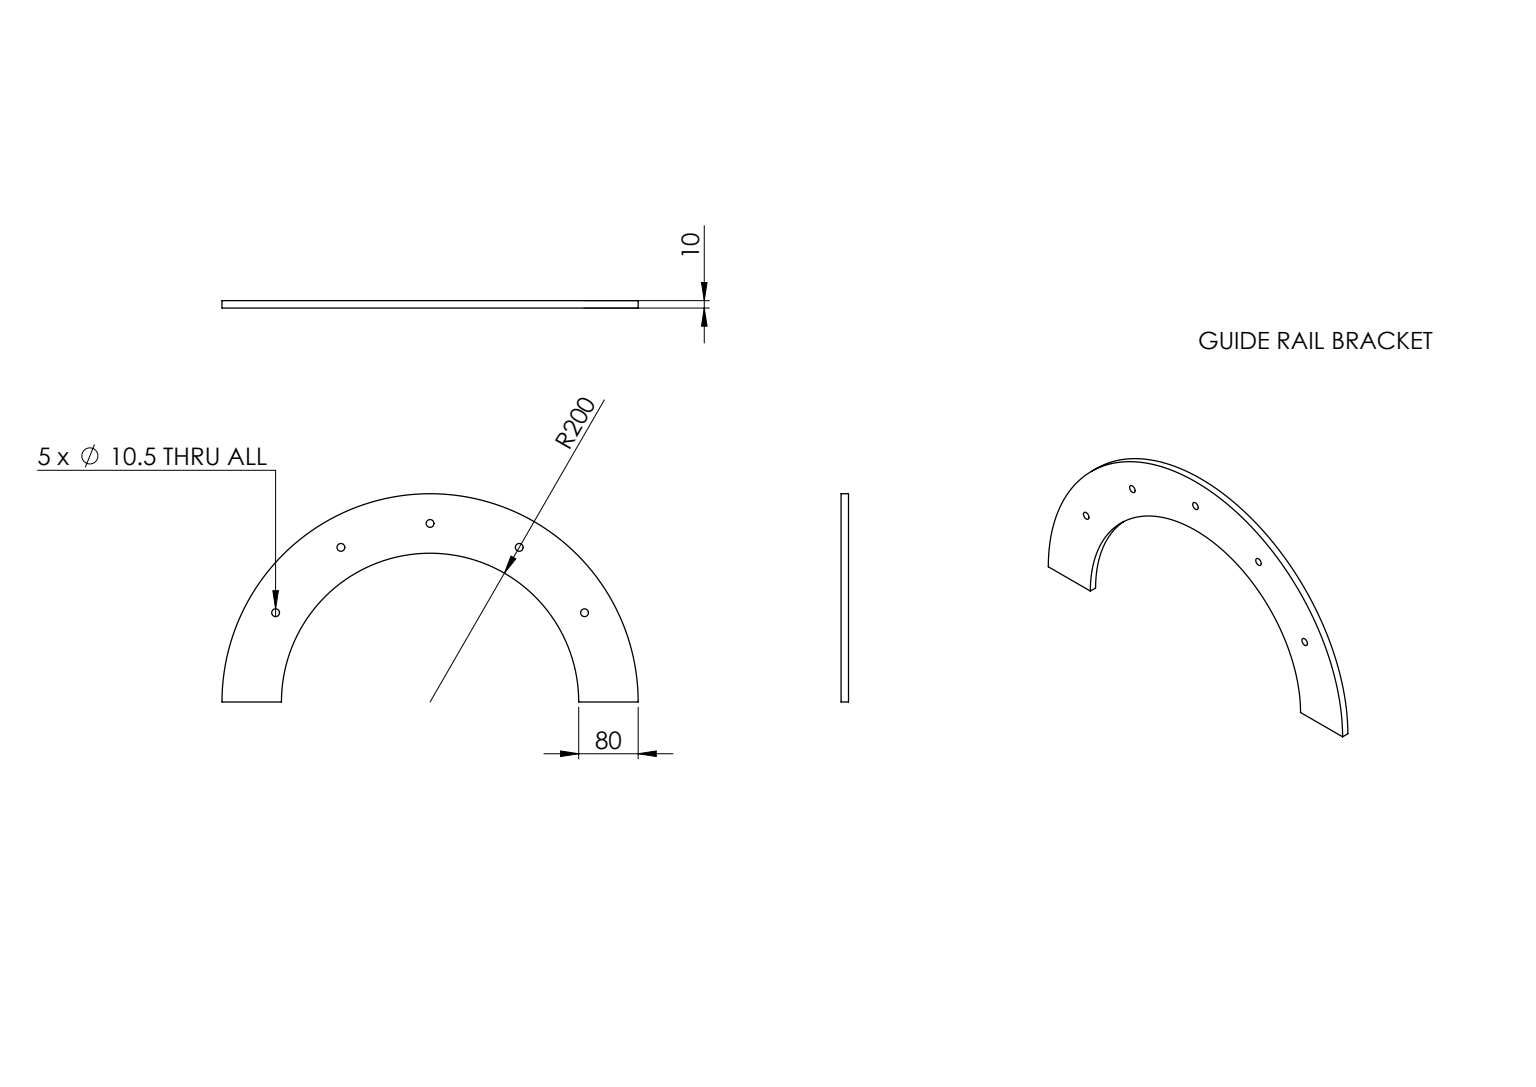
ISO-10303-21;
HEADER;
FILE_DESCRIPTION (('STEP AP214'),
    '1' );
FILE_NAME ('Guide Rail Bracket.step',
    '2026-10-23T05:12:30',
    ( '' ),
    ( '' ),
    'SwSTEP 2.0',
    'SolidWorks 2026',
    '' );
FILE_SCHEMA (( 'AUTOMOTIVE_DESIGN' ));
ENDSEC;

DATA;
#10=CARTESIAN_POINT ( 'NONE',  ( 213.0929183184020701, 119.9981648402868331, 10.00000000000000000 ) ) ;
#18=CARTESIAN_POINT ( 'NONE',  ( -5.249999999999968026, 239.9963296805737230, 10.00000000000000000 ) ) ;
#20=DIRECTION ( 'NONE',  ( -1.000000000000000000, 0.000000000000000000, 0.000000000000000000 ) ) ;
#21=CARTESIAN_POINT ( 'NONE',  ( -279.9963296805736945, 3.428966089163216048E-14, 0.000000000000000000 ) ) ;
#25=DIRECTION ( 'NONE',  ( -0.000000000000000000, -0.000000000000000000, 1.000000000000000000 ) ) ;
#29=DIRECTION ( 'NONE',  ( -1.000000000000000000, 0.000000000000000000, 0.000000000000000000 ) ) ;
#37=CIRCLE ( 'NONE', #2942, 5.249999999999991118 ) ;
#54=FACE_BOUND ( 'NONE', #7641, .T. ) ;
#72=ORIENTED_EDGE ( 'NONE', *, *, #191, .F. ) ;
#80=ORIENTED_EDGE ( 'NONE', *, *, #2127, .F. ) ;
#86=CARTESIAN_POINT ( 'NONE',  ( 1.469553684752138043E-14, 239.9963296805737230, 10.00000000000000178 ) ) ;
#121=CARTESIAN_POINT ( 'NONE',  ( -125.2481648402867762, 207.8429183184021554, -8.673617379884035472E-15 ) ) ;
#157=VECTOR ( 'NONE', #4793, 1000.000000000000000 ) ;
#162=DIRECTION ( 'NONE',  ( -0.000000000000000000, -0.000000000000000000, 1.000000000000000000 ) ) ;
#172=ORIENTED_EDGE ( 'NONE', *, *, #2324, .T. ) ;
#173=AXIS2_PLACEMENT_3D ( 'NONE', #1594, #994, #5732 ) ;
#191=EDGE_CURVE ( 'NONE', #6189, #4002, #7244, .T. ) ;
#198=AXIS2_PLACEMENT_3D ( 'NONE', #1671, #7152, #4070 ) ;
#201=DIRECTION ( 'NONE',  ( -2.403401228516536951E-14, -1.000000000000000000, 0.000000000000000000 ) ) ;
#272=ORIENTED_EDGE ( 'NONE', *, *, #7163, .T. ) ;
#285=CARTESIAN_POINT ( 'NONE',  ( -207.8429183184020985, 119.9981648402869467, 10.00000000000000178 ) ) ;
#298=CIRCLE ( 'NONE', #1308, 5.249999999999976907 ) ;
#311=CARTESIAN_POINT ( 'NONE',  ( 202.5929183184021269, 119.9981648402868331, 10.00000000000000000 ) ) ;
#315=EDGE_CURVE ( 'NONE', #1373, #3431, #4733, .T. ) ;
#334=ORIENTED_EDGE ( 'NONE', *, *, #2127, .T. ) ;
#346=DIRECTION ( 'NONE',  ( 1.000000000000000000, 0.000000000000000000, 0.000000000000000000 ) ) ;
#360=ORIENTED_EDGE ( 'NONE', *, *, #6201, .F. ) ;
#372=EDGE_LOOP ( 'NONE', ( #1862, #4014 ) ) ;
#378=CARTESIAN_POINT ( 'NONE',  ( -279.9963296805736945, 3.428966089163216048E-14, 10.00000000000000000 ) ) ;
#384=DIRECTION ( 'NONE',  ( -0.000000000000000000, -0.000000000000000000, 1.000000000000000000 ) ) ;
#389=DIRECTION ( 'NONE',  ( -0.000000000000000000, -0.000000000000000000, 1.000000000000000000 ) ) ;
#411=EDGE_CURVE ( 'NONE', #2919, #6189, #1551, .T. ) ;
#423=AXIS2_PLACEMENT_3D ( 'NONE', #6991, #7495, #3952 ) ;
#425=CARTESIAN_POINT ( 'NONE',  ( 119.9981648402868899, 207.8429183184021269, 10.00000000000000000 ) ) ;
#431=ORIENTED_EDGE ( 'NONE', *, *, #935, .T. ) ;
#492=ORIENTED_EDGE ( 'NONE', *, *, #2605, .F. ) ;
#551=ORIENTED_EDGE ( 'NONE', *, *, #3232, .F. ) ;
#557=AXIS2_PLACEMENT_3D ( 'NONE', #5104, #4513, #3373 ) ;
#560=EDGE_CURVE ( 'NONE', #7291, #3873, #1586, .T. ) ;
#594=ORIENTED_EDGE ( 'NONE', *, *, #7692, .T. ) ;
#598=DIRECTION ( 'NONE',  ( 1.000000000000000000, 0.000000000000000000, 0.000000000000000000 ) ) ;
#622=DIRECTION ( 'NONE',  ( 1.000000000000000000, 0.000000000000000000, 0.000000000000000000 ) ) ;
#651=DIRECTION ( 'NONE',  ( -0.000000000000000000, -0.000000000000000000, 1.000000000000000000 ) ) ;
#673=DIRECTION ( 'NONE',  ( -1.000000000000000000, 0.000000000000000000, 0.000000000000000000 ) ) ;
#675=CARTESIAN_POINT ( 'NONE',  ( -279.9963296805736945, 3.428966089163216048E-14, 10.00000000000000000 ) ) ;
#690=DIRECTION ( 'NONE',  ( 1.000000000000000000, 0.000000000000000000, 0.000000000000000000 ) ) ;
#710=ORIENTED_EDGE ( 'NONE', *, *, #4511, .F. ) ;
#712=ADVANCED_FACE ( 'NONE', ( #6130 ), #4936, .T. ) ;
#730=CYLINDRICAL_SURFACE ( 'NONE', #6902, 5.249999999999983125 ) ;
#735=ORIENTED_EDGE ( 'NONE', *, *, #1621, .F. ) ;
#745=ORIENTED_EDGE ( 'NONE', *, *, #3810, .T. ) ;
#774=EDGE_LOOP ( 'NONE', ( #3751, #5530 ) ) ;
#785=DIRECTION ( 'NONE',  ( -0.000000000000000000, -0.000000000000000000, 1.000000000000000000 ) ) ;
#800=CIRCLE ( 'NONE', #1055, 5.249999999999976907 ) ;
#808=COLOUR_RGB ( '',0.8941176470588234615, 0.8941176470588234615, 0.8941176470588234615 ) ;
#813=ORIENTED_EDGE ( 'NONE', *, *, #1830, .T. ) ;
#828=FILL_AREA_STYLE ('',( #863 ) ) ;
#852=ADVANCED_FACE ( 'NONE', ( #869 ), #3838, .T. ) ;
#863=FILL_AREA_STYLE_COLOUR ( '', #808 ) ;
#869=FACE_OUTER_BOUND ( 'NONE', #5970, .T. ) ;
#887=VERTEX_POINT ( 'NONE', #3911 ) ;
#893=DIRECTION ( 'NONE',  ( -0.000000000000000000, -0.000000000000000000, 1.000000000000000000 ) ) ;
#904=ORIENTED_EDGE ( 'NONE', *, *, #5478, .F. ) ;
#913=VERTEX_POINT ( 'NONE', #2307 ) ;
#935=EDGE_CURVE ( 'NONE', #887, #5491, #2493, .T. ) ;
#943=DIRECTION ( 'NONE',  ( 1.000000000000000000, 0.000000000000000000, 0.000000000000000000 ) ) ;
#994=DIRECTION ( 'NONE',  ( -0.000000000000000000, -0.000000000000000000, -1.000000000000000000 ) ) ;
#999=EDGE_LOOP ( 'NONE', ( #3310, #3719, #5793, #4925 ) ) ;
#1050=DIRECTION ( 'NONE',  ( -0.000000000000000000, -0.000000000000000000, 1.000000000000000000 ) ) ;
#1055=AXIS2_PLACEMENT_3D ( 'NONE', #2477, #1994, #6680 ) ;
#1063=EDGE_LOOP ( 'NONE', ( #4829, #3062, #2505, #4842 ) ) ;
#1069=FACE_OUTER_BOUND ( 'NONE', #6626, .T. ) ;
#1075=CARTESIAN_POINT ( 'NONE',  ( -119.9981648402868046, 207.8429183184021554, -8.673617379884035472E-15 ) ) ;
#1100=FACE_BOUND ( 'NONE', #7449, .T. ) ;
#1130=ORIENTED_EDGE ( 'NONE', *, *, #6583, .T. ) ;
#1131=ORIENTED_EDGE ( 'NONE', *, *, #5478, .T. ) ;
#1182=ORIENTED_EDGE ( 'NONE', *, *, #6944, .T. ) ;
#1187=AXIS2_PLACEMENT_3D ( 'NONE', #1075, #5935, #4073 ) ;
#1190=ORIENTED_EDGE ( 'NONE', *, *, #3670, .T. ) ;
#1203=ORIENTED_EDGE ( 'NONE', *, *, #2453, .F. ) ;
#1222=AXIS2_PLACEMENT_3D ( 'NONE', #2444, #7326, #5503 ) ;
#1223=PRODUCT_DEFINITION ( 'UNKNOWN', '', #2441, #6530 ) ;
#1245=CARTESIAN_POINT ( 'NONE',  ( 1.469553684752138043E-14, 239.9963296805737230, 10.00000000000000000 ) ) ;
#1263=DIRECTION ( 'NONE',  ( -0.000000000000000000, -0.000000000000000000, -1.000000000000000000 ) ) ;
#1298=VERTEX_POINT ( 'NONE', #2939 ) ;
#1301=CARTESIAN_POINT ( 'NONE',  ( 0.000000000000000000, 0.000000000000000000, 0.000000000000000000 ) ) ;
#1308=AXIS2_PLACEMENT_3D ( 'NONE', #285, #6411, #2158 ) ;
#1341=LINE ( 'NONE', #675, #2511 ) ;
#1373=VERTEX_POINT ( 'NONE', #5397 ) ;
#1379=( NAMED_UNIT ( * ) PLANE_ANGLE_UNIT ( ) SI_UNIT ( $, .RADIAN. ) );
#1411=AXIS2_PLACEMENT_3D ( 'NONE', #86, #7191, #2390 ) ;
#1474=ADVANCED_FACE ( 'NONE', ( #1733 ), #4045, .F. ) ;
#1490=CIRCLE ( 'NONE', #6533, 5.249999999999976907 ) ;
#1498=SURFACE_STYLE_FILL_AREA ( #828 ) ;
#1518=ADVANCED_FACE ( 'NONE', ( #6141 ), #730, .F. ) ;
#1523=ADVANCED_FACE ( 'NONE', ( #7396 ), #3655, .F. ) ;
#1536=SHAPE_REPRESENTATION_RELATIONSHIP ( 'NONE' , 'NONE' ,  #5768, #1719 ) ;
#1539=DIRECTION ( 'NONE',  ( 1.000000000000000000, 2.398081733190338127E-14, 0.000000000000000000 ) ) ;
#1543=DIRECTION ( 'NONE',  ( -0.000000000000000000, -0.000000000000000000, 1.000000000000000000 ) ) ;
#1547=CYLINDRICAL_SURFACE ( 'NONE', #6081, 5.249999999999976907 ) ;
#1551=LINE ( 'NONE', #5140, #1712 ) ;
#1560=ORIENTED_EDGE ( 'NONE', *, *, #7226, .F. ) ;
#1574=DIRECTION ( 'NONE',  ( -0.000000000000000000, -0.000000000000000000, 1.000000000000000000 ) ) ;
#1582=VERTEX_POINT ( 'NONE', #3732 ) ;
#1586=CIRCLE ( 'NONE', #198, 5.249999999999976907 ) ;
#1594=CARTESIAN_POINT ( 'NONE',  ( 0.000000000000000000, 0.000000000000000000, 0.000000000000000000 ) ) ;
#1609=VERTEX_POINT ( 'NONE', #5430 ) ;
#1615=VECTOR ( 'NONE', #25, 1000.000000000000000 ) ;
#1618=EDGE_LOOP ( 'NONE', ( #1560, #2255, #813, #2345 ) ) ;
#1621=EDGE_CURVE ( 'NONE', #3939, #3350, #6218, .T. ) ;
#1641=AXIS2_PLACEMENT_3D ( 'NONE', #3794, #6045, #3674 ) ;
#1671=CARTESIAN_POINT ( 'NONE',  ( -207.8429183184020985, 119.9981648402869467, -8.673617379884035472E-15 ) ) ;
#1680=ORIENTED_EDGE ( 'NONE', *, *, #7692, .F. ) ;
#1687=AXIS2_PLACEMENT_3D ( 'NONE', #5556, #1936, #1859 ) ;
#1701=DIRECTION ( 'NONE',  ( -0.000000000000000000, 0.000000000000000000, -1.000000000000000000 ) ) ;
#1712=VECTOR ( 'NONE', #6252, 1000.000000000000000 ) ;
#1719=ADVANCED_BREP_SHAPE_REPRESENTATION ( '', ( #3160, #7485 ), #7608 ) ;
#1733=FACE_OUTER_BOUND ( 'NONE', #5351, .T. ) ;
#1737=ORIENTED_EDGE ( 'NONE', *, *, #2729, .F. ) ;
#1774=DIRECTION ( 'NONE',  ( -0.000000000000000000, -0.000000000000000000, 1.000000000000000000 ) ) ;
#1784=CARTESIAN_POINT ( 'NONE',  ( -213.0929183184020701, 119.9981648402869467, -8.673617379884035472E-15 ) ) ;
#1799=DIRECTION ( 'NONE',  ( -0.000000000000000000, -0.000000000000000000, -1.000000000000000000 ) ) ;
#1830=EDGE_CURVE ( 'NONE', #1298, #1609, #4113, .T. ) ;
#1859=DIRECTION ( 'NONE',  ( 1.000000000000000000, 0.000000000000000000, 0.000000000000000000 ) ) ;
#1862=ORIENTED_EDGE ( 'NONE', *, *, #315, .F. ) ;
#1895=( LENGTH_UNIT ( ) NAMED_UNIT ( * ) SI_UNIT ( .MILLI., .METRE. ) );
#1910=DIRECTION ( 'NONE',  ( -0.000000000000000000, -0.000000000000000000, 1.000000000000000000 ) ) ;
#1929=EDGE_CURVE ( 'NONE', #5275, #2430, #5638, .T. ) ;
#1936=DIRECTION ( 'NONE',  ( -0.000000000000000000, -0.000000000000000000, 1.000000000000000000 ) ) ;
#1950=CIRCLE ( 'NONE', #557, 5.249999999999977796 ) ;
#1953=FACE_OUTER_BOUND ( 'NONE', #3916, .T. ) ;
#1975=ADVANCED_FACE ( 'NONE', ( #3140, #3178, #54, #7239, #6173, #6648 ), #4270, .T. ) ;
#1980=CARTESIAN_POINT ( 'NONE',  ( -199.9963296805737230, 0.000000000000000000, 0.000000000000000000 ) ) ;
#1994=DIRECTION ( 'NONE',  ( -0.000000000000000000, -0.000000000000000000, 1.000000000000000000 ) ) ;
#2008=AXIS2_PLACEMENT_3D ( 'NONE', #6798, #785, #2652 ) ;
#2063=( NAMED_UNIT ( * ) SI_UNIT ( $, .STERADIAN. ) SOLID_ANGLE_UNIT ( ) );
#2097=DIRECTION ( 'NONE',  ( 1.000000000000000000, 2.398081733190338127E-14, 0.000000000000000000 ) ) ;
#2098=CLOSED_SHELL ( 'NONE', ( #2595, #3549, #7539, #2215, #6494, #3606, #852, #5190, #712, #7026, #1975, #5173, #1523, #1518, #3847, #1474 ) ) ;
#2127=EDGE_CURVE ( 'NONE', #2919, #6450, #6804, .T. ) ;
#2130=ORIENTED_EDGE ( 'NONE', *, *, #5621, .F. ) ;
#2137=CARTESIAN_POINT ( 'NONE',  ( 114.7481648402869041, 207.8429183184021269, 10.00000000000000000 ) ) ;
#2143=SURFACE_STYLE_USAGE ( .BOTH. , #5641 ) ;
#2156=AXIS2_PLACEMENT_3D ( 'NONE', #5561, #1263, #673 ) ;
#2158=DIRECTION ( 'NONE',  ( 1.000000000000000000, 0.000000000000000000, 0.000000000000000000 ) ) ;
#2173=DIRECTION ( 'NONE',  ( -0.000000000000000000, -0.000000000000000000, 1.000000000000000000 ) ) ;
#2181=CARTESIAN_POINT ( 'NONE',  ( 119.9981648402868899, 207.8429183184021269, 10.00000000000000178 ) ) ;
#2215=ADVANCED_FACE ( 'NONE', ( #7425 ), #4980, .F. ) ;
#2244=EDGE_LOOP ( 'NONE', ( #431, #1190 ) ) ;
#2246=ORIENTED_EDGE ( 'NONE', *, *, #411, .T. ) ;
#2254=AXIS2_PLACEMENT_3D ( 'NONE', #3570, #3998, #5301 ) ;
#2255=ORIENTED_EDGE ( 'NONE', *, *, #5817, .F. ) ;
#2257=EDGE_LOOP ( 'NONE', ( #3728, #3351 ) ) ;
#2294=ORIENTED_EDGE ( 'NONE', *, *, #5817, .T. ) ;
#2304=ORIENTED_EDGE ( 'NONE', *, *, #5352, .T. ) ;
#2307=CARTESIAN_POINT ( 'NONE',  ( -202.5929183184021269, 119.9981648402869467, 10.00000000000000178 ) ) ;
#2314=EDGE_CURVE ( 'NONE', #3873, #7291, #1490, .T. ) ;
#2319=VECTOR ( 'NONE', #5125, 1000.000000000000000 ) ;
#2324=EDGE_CURVE ( 'NONE', #5401, #6223, #3520, .T. ) ;
#2328=CIRCLE ( 'NONE', #4195, 199.9963296805737230 ) ;
#2341=LINE ( 'NONE', #6431, #5297 ) ;
#2345=ORIENTED_EDGE ( 'NONE', *, *, #4700, .T. ) ;
#2351=ORIENTED_EDGE ( 'NONE', *, *, #6649, .T. ) ;
#2382=CYLINDRICAL_SURFACE ( 'NONE', #2817, 279.9963296805736945 ) ;
#2390=DIRECTION ( 'NONE',  ( 1.000000000000000000, 0.000000000000000000, 0.000000000000000000 ) ) ;
#2397=LINE ( 'NONE', #3681, #3896 ) ;
#2424=ORIENTED_EDGE ( 'NONE', *, *, #4511, .T. ) ;
#2430=VERTEX_POINT ( 'NONE', #3012 ) ;
#2441=PRODUCT_DEFINITION_FORMATION_WITH_SPECIFIED_SOURCE ( 'ANY', '', #5672, .NOT_KNOWN. ) ;
#2444=CARTESIAN_POINT ( 'NONE',  ( -119.9981648402868046, 207.8429183184021554, 10.00000000000000000 ) ) ;
#2453=EDGE_CURVE ( 'NONE', #3350, #6223, #1341, .T. ) ;
#2464=AXIS2_PLACEMENT_3D ( 'NONE', #2732, #389, #5053 ) ;
#2472=ORIENTED_EDGE ( 'NONE', *, *, #3571, .F. ) ;
#2477=CARTESIAN_POINT ( 'NONE',  ( 207.8429183184020985, 119.9981648402868331, 10.00000000000000178 ) ) ;
#2493=CIRCLE ( 'NONE', #6891, 5.249999999999976907 ) ;
#2505=ORIENTED_EDGE ( 'NONE', *, *, #7355, .T. ) ;
#2511=VECTOR ( 'NONE', #5449, 1000.000000000000000 ) ;
#2516=EDGE_LOOP ( 'NONE', ( #1680, #6600, #2351, #7054 ) ) ;
#2578=CYLINDRICAL_SURFACE ( 'NONE', #1641, 5.249999999999976907 ) ;
#2579=DIRECTION ( 'NONE',  ( -0.000000000000000000, -0.000000000000000000, -1.000000000000000000 ) ) ;
#2592=EDGE_CURVE ( 'NONE', #7016, #4741, #2758, .T. ) ;
#2595=ADVANCED_FACE ( 'NONE', ( #4607 ), #4645, .F. ) ;
#2605=EDGE_CURVE ( 'NONE', #6450, #4002, #3871, .T. ) ;
#2619=DIRECTION ( 'NONE',  ( 1.000000000000000000, -2.403401228516536951E-14, 0.000000000000000000 ) ) ;
#2652=DIRECTION ( 'NONE',  ( 1.000000000000000000, 0.000000000000000000, 0.000000000000000000 ) ) ;
#2670=DIRECTION ( 'NONE',  ( 1.000000000000000000, 0.000000000000000000, 0.000000000000000000 ) ) ;
#2671=ORIENTED_EDGE ( 'NONE', *, *, #4700, .F. ) ;
#2674=ORIENTED_EDGE ( 'NONE', *, *, #7409, .T. ) ;
#2677=CARTESIAN_POINT ( 'NONE',  ( -114.7481648402868188, 207.8429183184021554, 10.00000000000000000 ) ) ;
#2682=ORIENTED_EDGE ( 'NONE', *, *, #6924, .T. ) ;
#2709=CIRCLE ( 'NONE', #1187, 5.249999999999976907 ) ;
#2729=EDGE_CURVE ( 'NONE', #7759, #7346, #4272, .T. ) ;
#2732=CARTESIAN_POINT ( 'NONE',  ( 119.9981648402868899, 207.8429183184021269, -8.673617379884035472E-15 ) ) ;
#2758=CIRCLE ( 'NONE', #7162, 5.249999999999976907 ) ;
#2767=LINE ( 'NONE', #311, #2319 ) ;
#2774=CIRCLE ( 'NONE', #5539, 5.249999999999976907 ) ;
#2795=APPLICATION_CONTEXT ( 'automotive_design' ) ;
#2817=AXIS2_PLACEMENT_3D ( 'NONE', #2965, #2884, #6591 ) ;
#2821=CARTESIAN_POINT ( 'NONE',  ( 5.249999999999997335, 239.9963296805737230, 10.00000000000000000 ) ) ;
#2841=ORIENTED_EDGE ( 'NONE', *, *, #2605, .T. ) ;
#2852=CARTESIAN_POINT ( 'NONE',  ( -207.8429183184020985, 119.9981648402869467, -8.673617379884035472E-15 ) ) ;
#2856=AXIS2_PLACEMENT_3D ( 'NONE', #5052, #201, #2619 ) ;
#2884=DIRECTION ( 'NONE',  ( -0.000000000000000000, -0.000000000000000000, -1.000000000000000000 ) ) ;
#2889=AXIS2_PLACEMENT_3D ( 'NONE', #4948, #4436, #6849 ) ;
#2894=CARTESIAN_POINT ( 'NONE',  ( 199.9963296805737230, -4.860399174643270382E-12, 10.00000000000000000 ) ) ;
#2919=VERTEX_POINT ( 'NONE', #6070 ) ;
#2939=CARTESIAN_POINT ( 'NONE',  ( 5.249999999999992895, 239.9963296805737230, -8.673617379884035472E-15 ) ) ;
#2942=AXIS2_PLACEMENT_3D ( 'NONE', #3014, #7231, #598 ) ;
#2947=ORIENTED_EDGE ( 'NONE', *, *, #1929, .T. ) ;
#2962=CARTESIAN_POINT ( 'NONE',  ( -199.9963296805737230, 0.000000000000000000, 10.00000000000000000 ) ) ;
#2965=CARTESIAN_POINT ( 'NONE',  ( 0.000000000000000000, 0.000000000000000000, 10.00000000000000000 ) ) ;
#2980=DIRECTION ( 'NONE',  ( -0.000000000000000000, -0.000000000000000000, 1.000000000000000000 ) ) ;
#3000=VECTOR ( 'NONE', #4515, 1000.000000000000000 ) ;
#3012=CARTESIAN_POINT ( 'NONE',  ( 125.2481648402868615, 207.8429183184021269, 10.00000000000000178 ) ) ;
#3014=CARTESIAN_POINT ( 'NONE',  ( -119.9981648402868046, 207.8429183184021554, 10.00000000000000178 ) ) ;
#3019=LINE ( 'NONE', #18, #5201 ) ;
#3023=CARTESIAN_POINT ( 'NONE',  ( -202.5929183184021269, 119.9981648402869467, 10.00000000000000000 ) ) ;
#3027=STYLED_ITEM('',(#7809),#3160);
#3037=FACE_BOUND ( 'NONE', #2257, .T. ) ;
#3048=EDGE_LOOP ( 'NONE', ( #7092, #492, #4325, #745 ) ) ;
#3057=LINE ( 'NONE', #4348, #5595 ) ;
#3062=ORIENTED_EDGE ( 'NONE', *, *, #2592, .F. ) ;
#3140=FACE_BOUND ( 'NONE', #2244, .T. ) ;
#3148=DIRECTION ( 'NONE',  ( 1.000000000000000000, 0.000000000000000000, 0.000000000000000000 ) ) ;
#3160=MANIFOLD_SOLID_BREP ( 'M10 Clearance Hole1', #2098 ) ;
#3178=FACE_BOUND ( 'NONE', #5070, .T. ) ;
#3230=ORIENTED_EDGE ( 'NONE', *, *, #6924, .F. ) ;
#3232=EDGE_CURVE ( 'NONE', #5609, #6843, #2774, .T. ) ;
#3239=AXIS2_PLACEMENT_3D ( 'NONE', #7348, #3565, #5975 ) ;
#3260=DIRECTION ( 'NONE',  ( -0.000000000000000000, -0.000000000000000000, 1.000000000000000000 ) ) ;
#3272=DIRECTION ( 'NONE',  ( -0.000000000000000000, -0.000000000000000000, 1.000000000000000000 ) ) ;
#3276=ORIENTED_EDGE ( 'NONE', *, *, #2314, .F. ) ;
#3278=MECHANICAL_DESIGN_GEOMETRIC_PRESENTATION_REPRESENTATION('',(#3027),#7426);
#3288=CARTESIAN_POINT ( 'NONE',  ( 279.9963296805736945, -6.783120157456498832E-12, 10.00000000000000000 ) ) ;
#3310=ORIENTED_EDGE ( 'NONE', *, *, #2324, .F. ) ;
#3336=CIRCLE ( 'NONE', #3591, 5.249999999999977796 ) ;
#3350=VERTEX_POINT ( 'NONE', #378 ) ;
#3351=ORIENTED_EDGE ( 'NONE', *, *, #5352, .F. ) ;
#3365=DIRECTION ( 'NONE',  ( 1.000000000000000000, 0.000000000000000000, 0.000000000000000000 ) ) ;
#3373=DIRECTION ( 'NONE',  ( 1.000000000000000000, 0.000000000000000000, 0.000000000000000000 ) ) ;
#3390=CIRCLE ( 'NONE', #4391, 5.249999999999976907 ) ;
#3431=VERTEX_POINT ( 'NONE', #6437 ) ;
#3474=CARTESIAN_POINT ( 'NONE',  ( 0.000000000000000000, 0.000000000000000000, 0.000000000000000000 ) ) ;
#3510=VECTOR ( 'NONE', #5926, 1000.000000000000000 ) ;
#3520=LINE ( 'NONE', #4660, #3510 ) ;
#3549=ADVANCED_FACE ( 'NONE', ( #3714 ), #2578, .F. ) ;
#3552=VERTEX_POINT ( 'NONE', #3756 ) ;
#3561=EDGE_CURVE ( 'NONE', #7346, #7759, #2709, .T. ) ;
#3565=DIRECTION ( 'NONE',  ( -4.286207611454020849E-16, -1.000000000000000000, 0.000000000000000000 ) ) ;
#3570=CARTESIAN_POINT ( 'NONE',  ( 119.9981648402868899, 207.8429183184021269, 10.00000000000000178 ) ) ;
#3571=EDGE_CURVE ( 'NONE', #887, #6843, #6634, .T. ) ;
#3580=CIRCLE ( 'NONE', #173, 199.9963296805737230 ) ;
#3591=AXIS2_PLACEMENT_3D ( 'NONE', #5626, #3260, #2670 ) ;
#3603=EDGE_LOOP ( 'NONE', ( #272, #80, #904, #735 ) ) ;
#3606=ADVANCED_FACE ( 'NONE', ( #4890 ), #4970, .F. ) ;
#3611=DIRECTION ( 'NONE',  ( -0.000000000000000000, -0.000000000000000000, 1.000000000000000000 ) ) ;
#3655=CYLINDRICAL_SURFACE ( 'NONE', #1222, 5.249999999999976907 ) ;
#3657=PRODUCT_DEFINITION_SHAPE ( 'NONE', 'NONE',  #1223 ) ;
#3665=AXIS2_PLACEMENT_3D ( 'NONE', #425, #384, #5795 ) ;
#3670=EDGE_CURVE ( 'NONE', #5491, #887, #6936, .T. ) ;
#3674=DIRECTION ( 'NONE',  ( 1.000000000000000000, 0.000000000000000000, 0.000000000000000000 ) ) ;
#3681=CARTESIAN_POINT ( 'NONE',  ( -213.0929183184020701, 119.9981648402869467, 10.00000000000000000 ) ) ;
#3687=AXIS2_PLACEMENT_3D ( 'NONE', #3474, #4536, #1539 ) ;
#3699=ORIENTED_EDGE ( 'NONE', *, *, #935, .F. ) ;
#3703=ORIENTED_EDGE ( 'NONE', *, *, #1929, .F. ) ;
#3714=FACE_OUTER_BOUND ( 'NONE', #4569, .T. ) ;
#3719=ORIENTED_EDGE ( 'NONE', *, *, #3810, .F. ) ;
#3728=ORIENTED_EDGE ( 'NONE', *, *, #7657, .F. ) ;
#3732=CARTESIAN_POINT ( 'NONE',  ( -5.249999999999972466, 239.9963296805737230, 10.00000000000000178 ) ) ;
#3751=ORIENTED_EDGE ( 'NONE', *, *, #3561, .T. ) ;
#3756=CARTESIAN_POINT ( 'NONE',  ( -5.249999999999962697, 239.9963296805737230, -8.673617379884035472E-15 ) ) ;
#3758=DIRECTION ( 'NONE',  ( 0.000000000000000000, 0.000000000000000000, 1.000000000000000000 ) ) ;
#3762=AXIS2_PLACEMENT_3D ( 'NONE', #4466, #7535, #3365 ) ;
#3794=CARTESIAN_POINT ( 'NONE',  ( 119.9981648402868899, 207.8429183184021269, 10.00000000000000000 ) ) ;
#3803=CARTESIAN_POINT ( 'NONE',  ( -114.7481648402868188, 207.8429183184021554, -8.673617379884035472E-15 ) ) ;
#3810=EDGE_CURVE ( 'NONE', #3939, #5401, #2341, .T. ) ;
#3838=PLANE ( 'NONE',  #2856 ) ;
#3847=ADVANCED_FACE ( 'NONE', ( #7178 ), #4051, .F. ) ;
#3854=CARTESIAN_POINT ( 'NONE',  ( -199.9963296805737230, 0.000000000000000000, 10.00000000000000000 ) ) ;
#3865=ORIENTED_EDGE ( 'NONE', *, *, #3232, .T. ) ;
#3871=LINE ( 'NONE', #6165, #6795 ) ;
#3873=VERTEX_POINT ( 'NONE', #1784 ) ;
#3889=SHAPE_DEFINITION_REPRESENTATION ( #3657, #5768 ) ;
#3892=ORIENTED_EDGE ( 'NONE', *, *, #7735, .F. ) ;
#3896=VECTOR ( 'NONE', #3611, 1000.000000000000000 ) ;
#3911=CARTESIAN_POINT ( 'NONE',  ( 213.0929183184020701, 119.9981648402868331, -8.673617379884035472E-15 ) ) ;
#3916=EDGE_LOOP ( 'NONE', ( #4402, #5080, #5549, #4519 ) ) ;
#3939=VERTEX_POINT ( 'NONE', #2962 ) ;
#3952=DIRECTION ( 'NONE',  ( 1.000000000000000000, 0.000000000000000000, 0.000000000000000000 ) ) ;
#3998=DIRECTION ( 'NONE',  ( -0.000000000000000000, -0.000000000000000000, 1.000000000000000000 ) ) ;
#4002=VERTEX_POINT ( 'NONE', #7295 ) ;
#4014=ORIENTED_EDGE ( 'NONE', *, *, #6583, .F. ) ;
#4045=CYLINDRICAL_SURFACE ( 'NONE', #7278, 5.249999999999976907 ) ;
#4051=CYLINDRICAL_SURFACE ( 'NONE', #3665, 5.249999999999976907 ) ;
#4070=DIRECTION ( 'NONE',  ( 1.000000000000000000, 0.000000000000000000, 0.000000000000000000 ) ) ;
#4073=DIRECTION ( 'NONE',  ( 1.000000000000000000, 0.000000000000000000, 0.000000000000000000 ) ) ;
#4113=LINE ( 'NONE', #2821, #6023 ) ;
#4194=CARTESIAN_POINT ( 'NONE',  ( 0.000000000000000000, 0.000000000000000000, 10.00000000000000000 ) ) ;
#4195=AXIS2_PLACEMENT_3D ( 'NONE', #4194, #1799, #4602 ) ;
#4203=CARTESIAN_POINT ( 'NONE',  ( -119.9981648402868046, 207.8429183184021554, 10.00000000000000178 ) ) ;
#4247=PLANE ( 'NONE',  #4572 ) ;
#4270=PLANE ( 'NONE',  #6147 ) ;
#4272=CIRCLE ( 'NONE', #4401, 5.249999999999976907 ) ;
#4294=( NAMED_UNIT ( * ) PLANE_ANGLE_UNIT ( ) SI_UNIT ( $, .RADIAN. ) );
#4325=ORIENTED_EDGE ( 'NONE', *, *, #7163, .F. ) ;
#4348=CARTESIAN_POINT ( 'NONE',  ( 125.2481648402868615, 207.8429183184021269, 10.00000000000000000 ) ) ;
#4353=AXIS2_PLACEMENT_3D ( 'NONE', #4203, #651, #690 ) ;
#4378=( NAMED_UNIT ( * ) PLANE_ANGLE_UNIT ( ) SI_UNIT ( $, .RADIAN. ) );
#4391=AXIS2_PLACEMENT_3D ( 'NONE', #2181, #6908, #6353 ) ;
#4401=AXIS2_PLACEMENT_3D ( 'NONE', #7171, #1050, #622 ) ;
#4402=ORIENTED_EDGE ( 'NONE', *, *, #4896, .F. ) ;
#4436=DIRECTION ( 'NONE',  ( -0.000000000000000000, -0.000000000000000000, 1.000000000000000000 ) ) ;
#4454=CIRCLE ( 'NONE', #1687, 5.249999999999976907 ) ;
#4459=CIRCLE ( 'NONE', #2464, 5.249999999999976907 ) ;
#4466=CARTESIAN_POINT ( 'NONE',  ( -119.9981648402868046, 207.8429183184021554, 10.00000000000000000 ) ) ;
#4480=ORIENTED_EDGE ( 'NONE', *, *, #411, .F. ) ;
#4489=CARTESIAN_POINT ( 'NONE',  ( 202.5929183184021269, 119.9981648402868331, -8.673617379884035472E-15 ) ) ;
#4496=DIRECTION ( 'NONE',  ( -0.000000000000000000, -0.000000000000000000, 1.000000000000000000 ) ) ;
#4511=EDGE_CURVE ( 'NONE', #7759, #3431, #5987, .T. ) ;
#4513=DIRECTION ( 'NONE',  ( -0.000000000000000000, -0.000000000000000000, 1.000000000000000000 ) ) ;
#4515=DIRECTION ( 'NONE',  ( -1.000000000000000000, 4.286207611454020849E-16, 0.000000000000000000 ) ) ;
#4516=CIRCLE ( 'NONE', #2889, 5.249999999999988454 ) ;
#4519=ORIENTED_EDGE ( 'NONE', *, *, #7657, .T. ) ;
#4536=DIRECTION ( 'NONE',  ( -0.000000000000000000, -0.000000000000000000, -1.000000000000000000 ) ) ;
#4539=CARTESIAN_POINT ( 'NONE',  ( 207.8429183184020985, 119.9981648402868331, -8.673617379884035472E-15 ) ) ;
#4569=EDGE_LOOP ( 'NONE', ( #6489, #7562, #2947, #6301 ) ) ;
#4572=AXIS2_PLACEMENT_3D ( 'NONE', #7330, #1701, #29 ) ;
#4573=CARTESIAN_POINT ( 'NONE',  ( 207.8429183184020985, 119.9981648402868331, -8.673617379884035472E-15 ) ) ;
#4602=DIRECTION ( 'NONE',  ( -1.000000000000000000, 0.000000000000000000, 0.000000000000000000 ) ) ;
#4607=FACE_OUTER_BOUND ( 'NONE', #6075, .T. ) ;
#4619=ORIENTED_EDGE ( 'NONE', *, *, #3670, .F. ) ;
#4635=ORIENTED_EDGE ( 'NONE', *, *, #4896, .T. ) ;
#4645=CYLINDRICAL_SURFACE ( 'NONE', #2008, 5.249999999999976907 ) ;
#4660=CARTESIAN_POINT ( 'NONE',  ( -199.9963296805737230, 0.000000000000000000, 0.000000000000000000 ) ) ;
#4700=EDGE_CURVE ( 'NONE', #1609, #1582, #4516, .T. ) ;
#4733=CIRCLE ( 'NONE', #4353, 5.249999999999991118 ) ;
#4741=VERTEX_POINT ( 'NONE', #5852 ) ;
#4759=CARTESIAN_POINT ( 'NONE',  ( -125.2481648402867762, 207.8429183184021554, 10.00000000000000000 ) ) ;
#4772=CARTESIAN_POINT ( 'NONE',  ( 114.7481648402869041, 207.8429183184021269, 10.00000000000000178 ) ) ;
#4793=DIRECTION ( 'NONE',  ( -1.000000000000000000, 2.403401228516536636E-14, 0.000000000000000000 ) ) ;
#4829=ORIENTED_EDGE ( 'NONE', *, *, #5486, .F. ) ;
#4837=FACE_BOUND ( 'NONE', #5628, .T. ) ;
#4841=( GEOMETRIC_REPRESENTATION_CONTEXT ( 3 ) GLOBAL_UNCERTAINTY_ASSIGNED_CONTEXT ( ( #6659 ) ) GLOBAL_UNIT_ASSIGNED_CONTEXT ( ( #6276, #1379, #2063 ) ) REPRESENTATION_CONTEXT ( 'NONE', 'WORKASPACE' ) );
#4842=ORIENTED_EDGE ( 'NONE', *, *, #5089, .T. ) ;
#4849=ORIENTED_EDGE ( 'NONE', *, *, #5089, .F. ) ;
#4890=FACE_OUTER_BOUND ( 'NONE', #3048, .T. ) ;
#4896=EDGE_CURVE ( 'NONE', #3873, #5664, #2397, .T. ) ;
#4918=AXIS2_PLACEMENT_3D ( 'NONE', #4573, #1574, #346 ) ;
#4925=ORIENTED_EDGE ( 'NONE', *, *, #2453, .T. ) ;
#4936=PLANE ( 'NONE',  #3239 ) ;
#4948=CARTESIAN_POINT ( 'NONE',  ( 1.469553684752138043E-14, 239.9963296805737230, 10.00000000000000178 ) ) ;
#4965=EDGE_LOOP ( 'NONE', ( #5035, #551 ) ) ;
#4970=CYLINDRICAL_SURFACE ( 'NONE', #2156, 199.9963296805737230 ) ;
#4980=CYLINDRICAL_SURFACE ( 'NONE', #3762, 5.249999999999976907 ) ;
#4994=ORIENTED_EDGE ( 'NONE', *, *, #2314, .T. ) ;
#5003=CARTESIAN_POINT ( 'NONE',  ( 202.5929183184021269, 119.9981648402868331, 10.00000000000000178 ) ) ;
#5035=ORIENTED_EDGE ( 'NONE', *, *, #7409, .F. ) ;
#5040=DIRECTION ( 'NONE',  ( -0.000000000000000000, -0.000000000000000000, -1.000000000000000000 ) ) ;
#5052=CARTESIAN_POINT ( 'NONE',  ( 279.9963296805736945, -6.783120157456498832E-12, 10.00000000000000000 ) ) ;
#5053=DIRECTION ( 'NONE',  ( 1.000000000000000000, 0.000000000000000000, 0.000000000000000000 ) ) ;
#5058=ORIENTED_EDGE ( 'NONE', *, *, #5621, .T. ) ;
#5070=EDGE_LOOP ( 'NONE', ( #6701, #5097 ) ) ;
#5073=DIRECTION ( 'NONE',  ( 1.000000000000000000, 0.000000000000000000, 0.000000000000000000 ) ) ;
#5080=ORIENTED_EDGE ( 'NONE', *, *, #560, .F. ) ;
#5082=CYLINDRICAL_SURFACE ( 'NONE', #7356, 5.249999999999976907 ) ;
#5089=EDGE_CURVE ( 'NONE', #2430, #5275, #3390, .T. ) ;
#5091=MECHANICAL_DESIGN_GEOMETRIC_PRESENTATION_REPRESENTATION('',(#5219),#4841);
#5097=ORIENTED_EDGE ( 'NONE', *, *, #7499, .T. ) ;
#5104=CARTESIAN_POINT ( 'NONE',  ( 1.469553684752138043E-14, 239.9963296805737230, -8.673617379884035472E-15 ) ) ;
#5118=ORIENTED_EDGE ( 'NONE', *, *, #191, .T. ) ;
#5125=DIRECTION ( 'NONE',  ( -0.000000000000000000, -0.000000000000000000, 1.000000000000000000 ) ) ;
#5140=CARTESIAN_POINT ( 'NONE',  ( 279.9963296805736945, -6.783120157456498832E-12, 10.00000000000000000 ) ) ;
#5171=CARTESIAN_POINT ( 'NONE',  ( -207.8429183184020985, 119.9981648402869467, 10.00000000000000000 ) ) ;
#5173=ADVANCED_FACE ( 'NONE', ( #1953 ), #5082, .F. ) ;
#5190=ADVANCED_FACE ( 'NONE', ( #7140 ), #2382, .T. ) ;
#5200=ORIENTED_EDGE ( 'NONE', *, *, #3561, .F. ) ;
#5201=VECTOR ( 'NONE', #2980, 1000.000000000000000 ) ;
#5210=DIRECTION ( 'NONE',  ( 1.000000000000000000, 0.000000000000000000, 0.000000000000000000 ) ) ;
#5219=STYLED_ITEM ( 'NONE', ( #7453 ), #1719 ) ;
#5223=DIRECTION ( 'NONE',  ( -0.000000000000000000, -0.000000000000000000, 1.000000000000000000 ) ) ;
#5275=VERTEX_POINT ( 'NONE', #4772 ) ;
#5297=VECTOR ( 'NONE', #7604, 1000.000000000000000 ) ;
#5301=DIRECTION ( 'NONE',  ( 1.000000000000000000, 0.000000000000000000, 0.000000000000000000 ) ) ;
#5351=EDGE_LOOP ( 'NONE', ( #6417, #3699, #6554, #2674 ) ) ;
#5352=EDGE_CURVE ( 'NONE', #5664, #913, #4454, .T. ) ;
#5397=CARTESIAN_POINT ( 'NONE',  ( -114.7481648402868188, 207.8429183184021554, 10.00000000000000178 ) ) ;
#5401=VERTEX_POINT ( 'NONE', #1980 ) ;
#5430=CARTESIAN_POINT ( 'NONE',  ( 5.250000000000002665, 239.9963296805737230, 10.00000000000000178 ) ) ;
#5435=CARTESIAN_POINT ( 'NONE',  ( 125.2481648402868615, 207.8429183184021269, -8.673617379884035472E-15 ) ) ;
#5440=ORIENTED_EDGE ( 'NONE', *, *, #315, .T. ) ;
#5449=DIRECTION ( 'NONE',  ( -0.000000000000000000, -0.000000000000000000, -1.000000000000000000 ) ) ;
#5478=EDGE_CURVE ( 'NONE', #3350, #2919, #7362, .T. ) ;
#5486=EDGE_CURVE ( 'NONE', #4741, #5275, #7408, .T. ) ;
#5491=VERTEX_POINT ( 'NONE', #4489 ) ;
#5503=DIRECTION ( 'NONE',  ( 1.000000000000000000, 0.000000000000000000, 0.000000000000000000 ) ) ;
#5530=ORIENTED_EDGE ( 'NONE', *, *, #2729, .T. ) ;
#5534=CARTESIAN_POINT ( 'NONE',  ( 0.000000000000000000, 0.000000000000000000, 0.000000000000000000 ) ) ;
#5539=AXIS2_PLACEMENT_3D ( 'NONE', #6423, #3272, #5073 ) ;
#5548=FACE_BOUND ( 'NONE', #372, .T. ) ;
#5549=ORIENTED_EDGE ( 'NONE', *, *, #6201, .T. ) ;
#5556=CARTESIAN_POINT ( 'NONE',  ( -207.8429183184020985, 119.9981648402869467, 10.00000000000000178 ) ) ;
#5561=CARTESIAN_POINT ( 'NONE',  ( 0.000000000000000000, 0.000000000000000000, 10.00000000000000000 ) ) ;
#5571=DIRECTION ( 'NONE',  ( -0.000000000000000000, 0.000000000000000000, -1.000000000000000000 ) ) ;
#5595=VECTOR ( 'NONE', #1910, 1000.000000000000000 ) ;
#5604=( NAMED_UNIT ( * ) SI_UNIT ( $, .STERADIAN. ) SOLID_ANGLE_UNIT ( ) );
#5609=VERTEX_POINT ( 'NONE', #5003 ) ;
#5621=EDGE_CURVE ( 'NONE', #7346, #1373, #5670, .T. ) ;
#5626=CARTESIAN_POINT ( 'NONE',  ( 1.469553684752138043E-14, 239.9963296805737230, -8.673617379884035472E-15 ) ) ;
#5628=EDGE_LOOP ( 'NONE', ( #2671, #6327 ) ) ;
#5638=CIRCLE ( 'NONE', #2254, 5.249999999999976907 ) ;
#5641=SURFACE_SIDE_STYLE ('',( #1498 ) ) ;
#5651=EDGE_LOOP ( 'NONE', ( #3892, #172, #2682, #5118 ) ) ;
#5664=VERTEX_POINT ( 'NONE', #7051 ) ;
#5670=LINE ( 'NONE', #2677, #7479 ) ;
#5672=PRODUCT ( 'Guide Rail Bracket', 'Guide Rail Bracket', '', ( #6889 ) ) ;
#5717=VECTOR ( 'NONE', #2173, 1000.000000000000000 ) ;
#5732=DIRECTION ( 'NONE',  ( -1.000000000000000000, 0.000000000000000000, 0.000000000000000000 ) ) ;
#5768=SHAPE_REPRESENTATION ( 'Guide Rail Bracket', ( #7485 ), #7608 ) ;
#5793=ORIENTED_EDGE ( 'NONE', *, *, #1621, .T. ) ;
#5795=DIRECTION ( 'NONE',  ( 1.000000000000000000, 0.000000000000000000, 0.000000000000000000 ) ) ;
#5800=VECTOR ( 'NONE', #6162, 1000.000000000000000 ) ;
#5817=EDGE_CURVE ( 'NONE', #1298, #3552, #3336, .T. ) ;
#5852=CARTESIAN_POINT ( 'NONE',  ( 114.7481648402869041, 207.8429183184021269, -8.673617379884035472E-15 ) ) ;
#5926=DIRECTION ( 'NONE',  ( -1.000000000000000000, 4.286207611454020849E-16, 0.000000000000000000 ) ) ;
#5935=DIRECTION ( 'NONE',  ( -0.000000000000000000, -0.000000000000000000, 1.000000000000000000 ) ) ;
#5949=VECTOR ( 'NONE', #6686, 1000.000000000000000 ) ;
#5970=EDGE_LOOP ( 'NONE', ( #72, #4480, #334, #2841 ) ) ;
#5975=DIRECTION ( 'NONE',  ( 1.000000000000000000, -4.286207611454020849E-16, 0.000000000000000000 ) ) ;
#5977=DIRECTION ( 'NONE',  ( 1.000000000000000000, 0.000000000000000000, 0.000000000000000000 ) ) ;
#5987=LINE ( 'NONE', #4759, #1615 ) ;
#5988=DIRECTION ( 'NONE',  ( 1.000000000000000000, 0.000000000000000000, 0.000000000000000000 ) ) ;
#6023=VECTOR ( 'NONE', #5223, 1000.000000000000000 ) ;
#6031=UNCERTAINTY_MEASURE_WITH_UNIT (LENGTH_MEASURE( 1.000000000000000082E-05 ), #7527, 'distance_accuracy_value', 'NONE');
#6045=DIRECTION ( 'NONE',  ( -0.000000000000000000, -0.000000000000000000, 1.000000000000000000 ) ) ;
#6070=CARTESIAN_POINT ( 'NONE',  ( 279.9963296805736945, -6.783120157456498832E-12, 10.00000000000000000 ) ) ;
#6075=EDGE_LOOP ( 'NONE', ( #4619, #1182, #3865, #2472 ) ) ;
#6081=AXIS2_PLACEMENT_3D ( 'NONE', #5171, #6476, #7574 ) ;
#6112=( NAMED_UNIT ( * ) SI_UNIT ( $, .STERADIAN. ) SOLID_ANGLE_UNIT ( ) );
#6125=CARTESIAN_POINT ( 'NONE',  ( 213.0929183184020701, 119.9981648402868331, 10.00000000000000178 ) ) ;
#6126=EDGE_LOOP ( 'NONE', ( #3230, #1203, #1131, #2246 ) ) ;
#6130=FACE_OUTER_BOUND ( 'NONE', #999, .T. ) ;
#6141=FACE_OUTER_BOUND ( 'NONE', #1618, .T. ) ;
#6145=FACE_BOUND ( 'NONE', #4965, .T. ) ;
#6147=AXIS2_PLACEMENT_3D ( 'NONE', #5534, #5571, #20 ) ;
#6162=DIRECTION ( 'NONE',  ( -0.000000000000000000, -0.000000000000000000, 1.000000000000000000 ) ) ;
#6165=CARTESIAN_POINT ( 'NONE',  ( 199.9963296805737230, -4.860399174643270382E-12, 10.00000000000000000 ) ) ;
#6173=FACE_BOUND ( 'NONE', #7376, .T. ) ;
#6189=VERTEX_POINT ( 'NONE', #7279 ) ;
#6201=EDGE_CURVE ( 'NONE', #7291, #913, #7201, .T. ) ;
#6218=LINE ( 'NONE', #3854, #3000 ) ;
#6223=VERTEX_POINT ( 'NONE', #21 ) ;
#6252=DIRECTION ( 'NONE',  ( -0.000000000000000000, -0.000000000000000000, -1.000000000000000000 ) ) ;
#6276=( LENGTH_UNIT ( ) NAMED_UNIT ( * ) SI_UNIT ( .MILLI., .METRE. ) );
#6301=ORIENTED_EDGE ( 'NONE', *, *, #7355, .F. ) ;
#6327=ORIENTED_EDGE ( 'NONE', *, *, #6649, .F. ) ;
#6345=CARTESIAN_POINT ( 'NONE',  ( 0.000000000000000000, 0.000000000000000000, 10.00000000000000000 ) ) ;
#6353=DIRECTION ( 'NONE',  ( 1.000000000000000000, 0.000000000000000000, 0.000000000000000000 ) ) ;
#6411=DIRECTION ( 'NONE',  ( -0.000000000000000000, -0.000000000000000000, 1.000000000000000000 ) ) ;
#6417=ORIENTED_EDGE ( 'NONE', *, *, #6944, .F. ) ;
#6423=CARTESIAN_POINT ( 'NONE',  ( 207.8429183184020985, 119.9981648402868331, 10.00000000000000178 ) ) ;
#6426=CARTESIAN_POINT ( 'NONE',  ( 119.9981648402868899, 207.8429183184021269, -8.673617379884035472E-15 ) ) ;
#6431=CARTESIAN_POINT ( 'NONE',  ( -199.9963296805737230, 0.000000000000000000, 10.00000000000000000 ) ) ;
#6437=CARTESIAN_POINT ( 'NONE',  ( -125.2481648402867762, 207.8429183184021554, 10.00000000000000178 ) ) ;
#6439=DIRECTION ( 'NONE',  ( 1.000000000000000000, 0.000000000000000000, 0.000000000000000000 ) ) ;
#6450=VERTEX_POINT ( 'NONE', #2894 ) ;
#6458=CIRCLE ( 'NONE', #1411, 5.249999999999988454 ) ;
#6476=DIRECTION ( 'NONE',  ( -0.000000000000000000, -0.000000000000000000, 1.000000000000000000 ) ) ;
#6489=ORIENTED_EDGE ( 'NONE', *, *, #7499, .F. ) ;
#6494=ADVANCED_FACE ( 'NONE', ( #1069 ), #1547, .F. ) ;
#6530=PRODUCT_DEFINITION_CONTEXT ( 'detailed design', #2795, 'design' ) ;
#6533=AXIS2_PLACEMENT_3D ( 'NONE', #2852, #7697, #6439 ) ;
#6539=CARTESIAN_POINT ( 'NONE',  ( 207.8429183184020985, 119.9981648402868331, 10.00000000000000000 ) ) ;
#6554=ORIENTED_EDGE ( 'NONE', *, *, #3571, .T. ) ;
#6566=CARTESIAN_POINT ( 'NONE',  ( -202.5929183184021269, 119.9981648402869467, -8.673617379884035472E-15 ) ) ;
#6583=EDGE_CURVE ( 'NONE', #3431, #1373, #37, .T. ) ;
#6591=DIRECTION ( 'NONE',  ( -1.000000000000000000, 0.000000000000000000, 0.000000000000000000 ) ) ;
#6600=ORIENTED_EDGE ( 'NONE', *, *, #7226, .T. ) ;
#6604=AXIS2_PLACEMENT_3D ( 'NONE', #6345, #5040, #2097 ) ;
#6611=UNCERTAINTY_MEASURE_WITH_UNIT (LENGTH_MEASURE( 1.000000000000000082E-05 ), #1895, 'distance_accuracy_value', 'NONE');
#6626=EDGE_LOOP ( 'NONE', ( #3276, #4635, #2304, #360 ) ) ;
#6634=LINE ( 'NONE', #10, #5800 ) ;
#6648=FACE_OUTER_BOUND ( 'NONE', #5651, .T. ) ;
#6649=EDGE_CURVE ( 'NONE', #1582, #1609, #6458, .T. ) ;
#6655=DIRECTION ( 'NONE',  ( -0.000000000000000000, -0.000000000000000000, 1.000000000000000000 ) ) ;
#6659=UNCERTAINTY_MEASURE_WITH_UNIT (LENGTH_MEASURE( 1.000000000000000082E-05 ), #6276, 'distance_accuracy_value', 'NONE');
#6680=DIRECTION ( 'NONE',  ( 1.000000000000000000, 0.000000000000000000, 0.000000000000000000 ) ) ;
#6686=DIRECTION ( 'NONE',  ( -0.000000000000000000, -0.000000000000000000, 1.000000000000000000 ) ) ;
#6689=CARTESIAN_POINT ( 'NONE',  ( 279.9963296805736945, -6.783120157456498832E-12, 0.000000000000000000 ) ) ;
#6701=ORIENTED_EDGE ( 'NONE', *, *, #2592, .T. ) ;
#6795=VECTOR ( 'NONE', #2579, 1000.000000000000000 ) ;
#6798=CARTESIAN_POINT ( 'NONE',  ( 207.8429183184020985, 119.9981648402868331, 10.00000000000000000 ) ) ;
#6804=LINE ( 'NONE', #3288, #7400 ) ;
#6838=CYLINDRICAL_SURFACE ( 'NONE', #423, 5.249999999999983125 ) ;
#6843=VERTEX_POINT ( 'NONE', #6125 ) ;
#6849=DIRECTION ( 'NONE',  ( 1.000000000000000000, 0.000000000000000000, 0.000000000000000000 ) ) ;
#6889=PRODUCT_CONTEXT ( 'NONE', #7419, 'mechanical' ) ;
#6891=AXIS2_PLACEMENT_3D ( 'NONE', #4539, #1543, #5210 ) ;
#6902=AXIS2_PLACEMENT_3D ( 'NONE', #1245, #6655, #3148 ) ;
#6908=DIRECTION ( 'NONE',  ( -0.000000000000000000, -0.000000000000000000, 1.000000000000000000 ) ) ;
#6924=EDGE_CURVE ( 'NONE', #6223, #6189, #7090, .T. ) ;
#6936=CIRCLE ( 'NONE', #4918, 5.249999999999976907 ) ;
#6944=EDGE_CURVE ( 'NONE', #5491, #5609, #2767, .T. ) ;
#6949=FACE_OUTER_BOUND ( 'NONE', #2516, .T. ) ;
#6991=CARTESIAN_POINT ( 'NONE',  ( 1.469553684752138043E-14, 239.9963296805737230, 10.00000000000000000 ) ) ;
#7016=VERTEX_POINT ( 'NONE', #5435 ) ;
#7026=ADVANCED_FACE ( 'NONE', ( #6145, #1100, #4837, #5548, #3037, #7251 ), #4247, .F. ) ;
#7051=CARTESIAN_POINT ( 'NONE',  ( -213.0929183184020701, 119.9981648402869467, 10.00000000000000178 ) ) ;
#7054=ORIENTED_EDGE ( 'NONE', *, *, #1830, .F. ) ;
#7090=CIRCLE ( 'NONE', #3687, 279.9963296805736945 ) ;
#7092=ORIENTED_EDGE ( 'NONE', *, *, #7735, .T. ) ;
#7140=FACE_OUTER_BOUND ( 'NONE', #6126, .T. ) ;
#7152=DIRECTION ( 'NONE',  ( -0.000000000000000000, -0.000000000000000000, 1.000000000000000000 ) ) ;
#7162=AXIS2_PLACEMENT_3D ( 'NONE', #6426, #162, #7638 ) ;
#7163=EDGE_CURVE ( 'NONE', #3939, #6450, #2328, .T. ) ;
#7171=CARTESIAN_POINT ( 'NONE',  ( -119.9981648402868046, 207.8429183184021554, -8.673617379884035472E-15 ) ) ;
#7175=EDGE_LOOP ( 'NONE', ( #1737, #2424, #1130, #2130 ) ) ;
#7178=FACE_OUTER_BOUND ( 'NONE', #1063, .T. ) ;
#7191=DIRECTION ( 'NONE',  ( -0.000000000000000000, -0.000000000000000000, 1.000000000000000000 ) ) ;
#7194=EDGE_LOOP ( 'NONE', ( #710, #5200, #5058, #5440 ) ) ;
#7201=LINE ( 'NONE', #3023, #5949 ) ;
#7226=EDGE_CURVE ( 'NONE', #3552, #1582, #3019, .T. ) ;
#7231=DIRECTION ( 'NONE',  ( -0.000000000000000000, -0.000000000000000000, 1.000000000000000000 ) ) ;
#7239=FACE_BOUND ( 'NONE', #774, .T. ) ;
#7244=LINE ( 'NONE', #6689, #157 ) ;
#7251=FACE_OUTER_BOUND ( 'NONE', #3603, .T. ) ;
#7278=AXIS2_PLACEMENT_3D ( 'NONE', #6539, #1774, #5988 ) ;
#7279=CARTESIAN_POINT ( 'NONE',  ( 279.9963296805736945, -6.783120157456498832E-12, 0.000000000000000000 ) ) ;
#7291=VERTEX_POINT ( 'NONE', #6566 ) ;
#7295=CARTESIAN_POINT ( 'NONE',  ( 199.9963296805737230, -4.860399174643270382E-12, 0.000000000000000000 ) ) ;
#7326=DIRECTION ( 'NONE',  ( -0.000000000000000000, -0.000000000000000000, 1.000000000000000000 ) ) ;
#7330=CARTESIAN_POINT ( 'NONE',  ( 0.000000000000000000, 0.000000000000000000, 10.00000000000000000 ) ) ;
#7346=VERTEX_POINT ( 'NONE', #3803 ) ;
#7348=CARTESIAN_POINT ( 'NONE',  ( -199.9963296805737230, 0.000000000000000000, 10.00000000000000000 ) ) ;
#7354=ORIENTED_EDGE ( 'NONE', *, *, #560, .T. ) ;
#7355=EDGE_CURVE ( 'NONE', #7016, #2430, #3057, .T. ) ;
#7356=AXIS2_PLACEMENT_3D ( 'NONE', #7489, #4496, #943 ) ;
#7362=CIRCLE ( 'NONE', #6604, 279.9963296805736945 ) ;
#7376=EDGE_LOOP ( 'NONE', ( #7354, #4994 ) ) ;
#7386=DIRECTION ( 'NONE',  ( -1.000000000000000000, 2.403401228516536636E-14, 0.000000000000000000 ) ) ;
#7396=FACE_OUTER_BOUND ( 'NONE', #7194, .T. ) ;
#7400=VECTOR ( 'NONE', #7386, 1000.000000000000000 ) ;
#7408=LINE ( 'NONE', #2137, #5717 ) ;
#7409=EDGE_CURVE ( 'NONE', #6843, #5609, #800, .T. ) ;
#7419=APPLICATION_CONTEXT ( 'automotive_design' ) ;
#7425=FACE_OUTER_BOUND ( 'NONE', #7175, .T. ) ;
#7426=( GEOMETRIC_REPRESENTATION_CONTEXT ( 3 ) GLOBAL_UNCERTAINTY_ASSIGNED_CONTEXT ( ( #6611 ) ) GLOBAL_UNIT_ASSIGNED_CONTEXT ( ( #1895, #4294, #6112 ) ) REPRESENTATION_CONTEXT ( 'NONE', 'WORKASPACE' ) );
#7449=EDGE_LOOP ( 'NONE', ( #4849, #3703 ) ) ;
#7453=PRESENTATION_STYLE_ASSIGNMENT (( #2143 ) ) ;
#7479=VECTOR ( 'NONE', #893, 1000.000000000000000 ) ;
#7485=AXIS2_PLACEMENT_3D ( 'NONE', #1301, #3758, #5977 ) ;
#7489=CARTESIAN_POINT ( 'NONE',  ( -207.8429183184020985, 119.9981648402869467, 10.00000000000000000 ) ) ;
#7495=DIRECTION ( 'NONE',  ( -0.000000000000000000, -0.000000000000000000, 1.000000000000000000 ) ) ;
#7499=EDGE_CURVE ( 'NONE', #4741, #7016, #4459, .T. ) ;
#7527=( LENGTH_UNIT ( ) NAMED_UNIT ( * ) SI_UNIT ( .MILLI., .METRE. ) );
#7535=DIRECTION ( 'NONE',  ( -0.000000000000000000, -0.000000000000000000, 1.000000000000000000 ) ) ;
#7539=ADVANCED_FACE ( 'NONE', ( #6949 ), #6838, .F. ) ;
#7562=ORIENTED_EDGE ( 'NONE', *, *, #5486, .T. ) ;
#7574=DIRECTION ( 'NONE',  ( 1.000000000000000000, 0.000000000000000000, 0.000000000000000000 ) ) ;
#7604=DIRECTION ( 'NONE',  ( -0.000000000000000000, -0.000000000000000000, -1.000000000000000000 ) ) ;
#7608=( GEOMETRIC_REPRESENTATION_CONTEXT ( 3 ) GLOBAL_UNCERTAINTY_ASSIGNED_CONTEXT ( ( #6031 ) ) GLOBAL_UNIT_ASSIGNED_CONTEXT ( ( #7527, #4378, #5604 ) ) REPRESENTATION_CONTEXT ( 'NONE', 'WORKASPACE' ) );
#7638=DIRECTION ( 'NONE',  ( 1.000000000000000000, 0.000000000000000000, 0.000000000000000000 ) ) ;
#7641=EDGE_LOOP ( 'NONE', ( #2294, #594 ) ) ;
#7657=EDGE_CURVE ( 'NONE', #913, #5664, #298, .T. ) ;
#7692=EDGE_CURVE ( 'NONE', #3552, #1298, #1950, .T. ) ;
#7697=DIRECTION ( 'NONE',  ( -0.000000000000000000, -0.000000000000000000, 1.000000000000000000 ) ) ;
#7735=EDGE_CURVE ( 'NONE', #5401, #4002, #3580, .T. ) ;
#7759=VERTEX_POINT ( 'NONE', #121 ) ;
#7803=COLOUR_RGB('Dark Blue',0.08,0.2,0.34);
#7804=FILL_AREA_STYLE_COLOUR('',#7803);
#7805=FILL_AREA_STYLE('',(#7804));
#7806=SURFACE_STYLE_FILL_AREA(#7805);
#7807=SURFACE_SIDE_STYLE('',(#7806));
#7808=SURFACE_STYLE_USAGE(.BOTH.,#7807);
#7809=PRESENTATION_STYLE_ASSIGNMENT((#7808));
ENDSEC;
END-ISO-10303-21;
